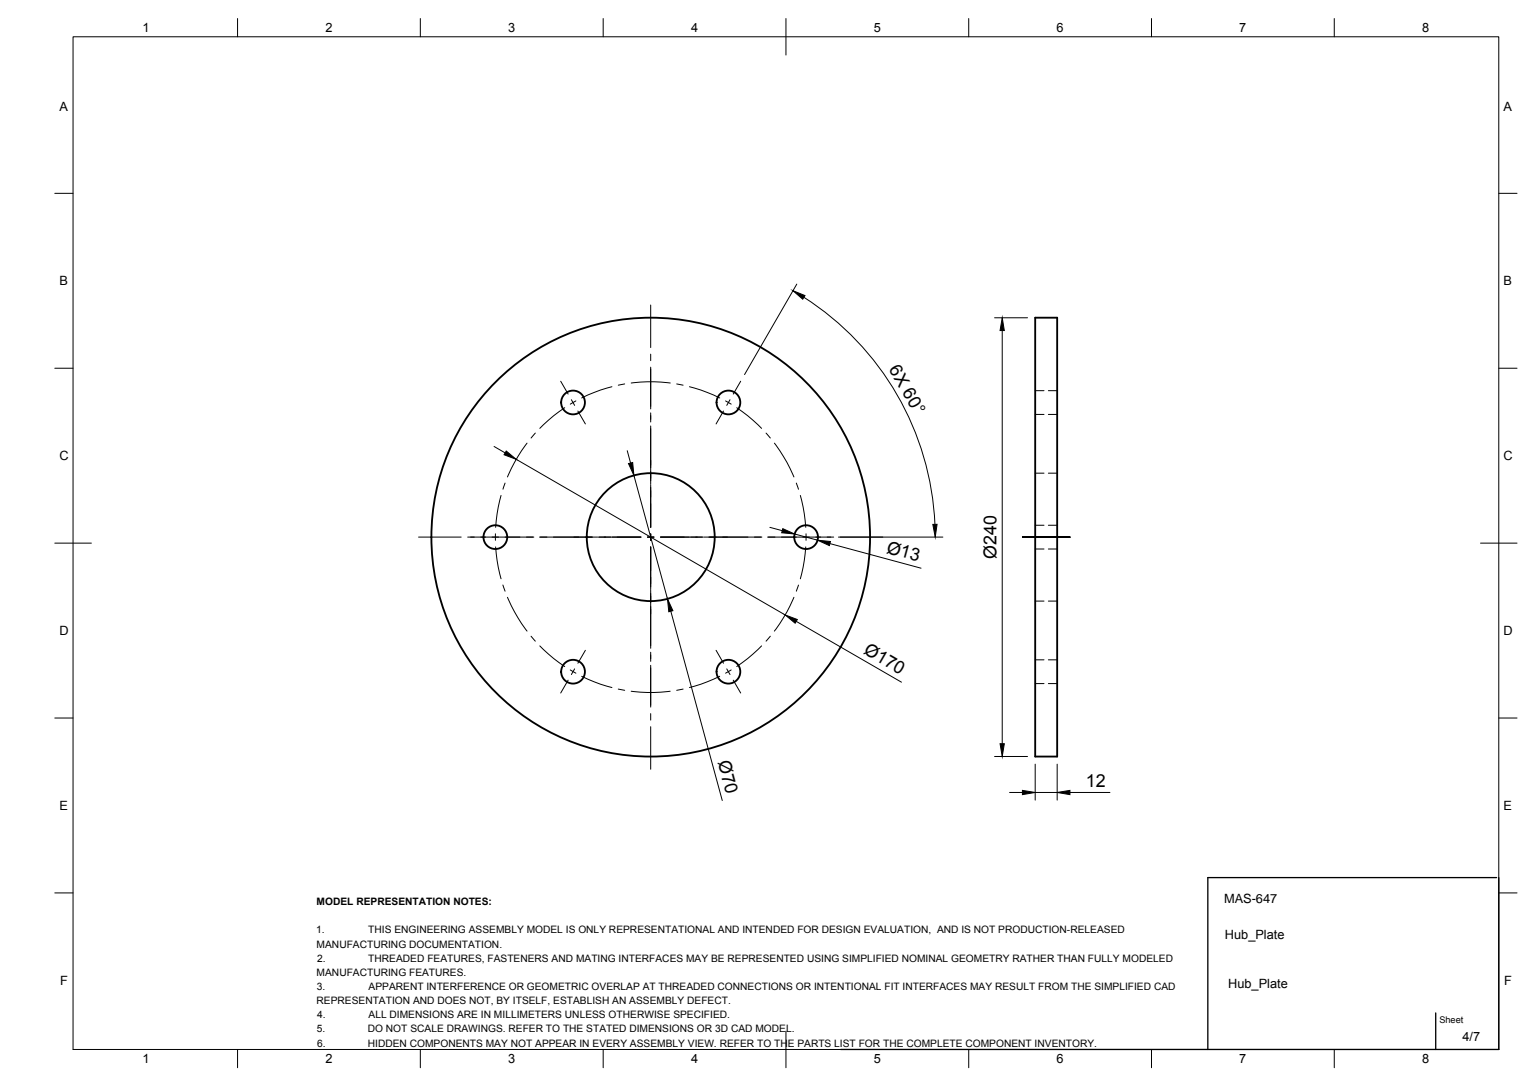
ISO-10303-21;
HEADER;
FILE_DESCRIPTION((''),'2;1');
FILE_NAME('Hub_Plate.step','2026-10-09T11:36:02-07:00',(''),(''),'','','');
FILE_SCHEMA (('AUTOMOTIVE_DESIGN { 1 0 10303 214 3 1 1 }'));
ENDSEC;
DATA;
#10=MECHANICAL_DESIGN_GEOMETRIC_PRESENTATION_REPRESENTATION('',(#83),#1549);
#73=SHAPE_REPRESENTATION_RELATIONSHIP('SRR','None',#1582,#78) ;
#78=ADVANCED_BREP_SHAPE_REPRESENTATION('',(#88),#1545) ;
#83=STYLED_ITEM('',(#1615),#88) ;
#88=MANIFOLD_SOLID_BREP('Body1',#845) ;
#106=FACE_BOUND('',#220,.T.) ;
#107=FACE_BOUND('',#221,.T.) ;
#108=FACE_BOUND('',#222,.T.) ;
#109=FACE_BOUND('',#223,.T.) ;
#110=FACE_BOUND('',#224,.T.) ;
#111=FACE_BOUND('',#225,.T.) ;
#112=FACE_BOUND('',#226,.T.) ;
#113=FACE_BOUND('',#228,.T.) ;
#114=FACE_BOUND('',#229,.T.) ;
#115=FACE_BOUND('',#230,.T.) ;
#116=FACE_BOUND('',#231,.T.) ;
#117=FACE_BOUND('',#232,.T.) ;
#118=FACE_BOUND('',#233,.T.) ;
#119=FACE_BOUND('',#234,.T.) ;
#125=PLANE('',#958) ;
#126=PLANE('',#959) ;
#151=FACE_OUTER_BOUND('',#211,.T.) ;
#152=FACE_OUTER_BOUND('',#212,.T.) ;
#153=FACE_OUTER_BOUND('',#213,.T.) ;
#154=FACE_OUTER_BOUND('',#214,.T.) ;
#155=FACE_OUTER_BOUND('',#215,.T.) ;
#156=FACE_OUTER_BOUND('',#216,.T.) ;
#157=FACE_OUTER_BOUND('',#217,.T.) ;
#158=FACE_OUTER_BOUND('',#218,.T.) ;
#159=FACE_OUTER_BOUND('',#219,.T.) ;
#160=FACE_OUTER_BOUND('',#227,.T.) ;
#211=EDGE_LOOP('',(#623,#624,#625,#626)) ;
#212=EDGE_LOOP('',(#627,#628,#629,#630)) ;
#213=EDGE_LOOP('',(#631,#632,#633,#634)) ;
#214=EDGE_LOOP('',(#635,#636,#637,#638)) ;
#215=EDGE_LOOP('',(#639,#640,#641,#642)) ;
#216=EDGE_LOOP('',(#643,#644,#645,#646)) ;
#217=EDGE_LOOP('',(#647,#648,#649,#650)) ;
#218=EDGE_LOOP('',(#651,#652,#653,#654)) ;
#219=EDGE_LOOP('',(#655)) ;
#220=EDGE_LOOP('',(#656)) ;
#221=EDGE_LOOP('',(#657)) ;
#222=EDGE_LOOP('',(#658)) ;
#223=EDGE_LOOP('',(#659)) ;
#224=EDGE_LOOP('',(#660)) ;
#225=EDGE_LOOP('',(#661)) ;
#226=EDGE_LOOP('',(#662)) ;
#227=EDGE_LOOP('',(#663)) ;
#228=EDGE_LOOP('',(#664)) ;
#229=EDGE_LOOP('',(#665)) ;
#230=EDGE_LOOP('',(#666)) ;
#231=EDGE_LOOP('',(#667)) ;
#232=EDGE_LOOP('',(#668)) ;
#233=EDGE_LOOP('',(#669)) ;
#234=EDGE_LOOP('',(#670)) ;
#272=LINE('',#1364,#320) ;
#273=LINE('',#1370,#321) ;
#274=LINE('',#1376,#322) ;
#275=LINE('',#1382,#323) ;
#276=LINE('',#1388,#324) ;
#277=LINE('',#1394,#325) ;
#278=LINE('',#1400,#326) ;
#279=LINE('',#1406,#327) ;
#320=VECTOR('',#1093,6.49999999999999) ;
#321=VECTOR('',#1100,6.49999999999999) ;
#322=VECTOR('',#1107,6.49999999999999) ;
#323=VECTOR('',#1114,6.49999999999999) ;
#324=VECTOR('',#1121,6.49999999999999) ;
#325=VECTOR('',#1128,6.49999999999999) ;
#326=VECTOR('',#1135,35.) ;
#327=VECTOR('',#1142,120.) ;
#376=CIRCLE('',#935,6.49999999999999) ;
#377=CIRCLE('',#936,6.49999999999999) ;
#378=CIRCLE('',#938,6.49999999999999) ;
#379=CIRCLE('',#939,6.49999999999998) ;
#380=CIRCLE('',#941,6.49999999999999) ;
#381=CIRCLE('',#942,6.49999999999999) ;
#382=CIRCLE('',#944,6.49999999999999) ;
#383=CIRCLE('',#945,6.49999999999999) ;
#384=CIRCLE('',#947,6.49999999999999) ;
#385=CIRCLE('',#948,6.49999999999999) ;
#386=CIRCLE('',#950,6.49999999999999) ;
#387=CIRCLE('',#951,6.49999999999999) ;
#388=CIRCLE('',#953,35.) ;
#389=CIRCLE('',#954,35.) ;
#390=CIRCLE('',#956,120.) ;
#391=CIRCLE('',#957,120.) ;
#428=VERTEX_POINT('',#1361) ;
#429=VERTEX_POINT('',#1363) ;
#430=VERTEX_POINT('',#1367) ;
#431=VERTEX_POINT('',#1369) ;
#432=VERTEX_POINT('',#1373) ;
#433=VERTEX_POINT('',#1375) ;
#434=VERTEX_POINT('',#1379) ;
#435=VERTEX_POINT('',#1381) ;
#436=VERTEX_POINT('',#1385) ;
#437=VERTEX_POINT('',#1387) ;
#438=VERTEX_POINT('',#1391) ;
#439=VERTEX_POINT('',#1393) ;
#440=VERTEX_POINT('',#1397) ;
#441=VERTEX_POINT('',#1399) ;
#442=VERTEX_POINT('',#1403) ;
#443=VERTEX_POINT('',#1405) ;
#499=EDGE_CURVE('',#428,#428,#376,.T.) ;
#500=EDGE_CURVE('',#428,#429,#272,.T.) ;
#501=EDGE_CURVE('',#429,#429,#377,.T.) ;
#502=EDGE_CURVE('',#430,#430,#378,.T.) ;
#503=EDGE_CURVE('',#430,#431,#273,.T.) ;
#504=EDGE_CURVE('',#431,#431,#379,.T.) ;
#505=EDGE_CURVE('',#432,#432,#380,.T.) ;
#506=EDGE_CURVE('',#432,#433,#274,.T.) ;
#507=EDGE_CURVE('',#433,#433,#381,.T.) ;
#508=EDGE_CURVE('',#434,#434,#382,.T.) ;
#509=EDGE_CURVE('',#434,#435,#275,.T.) ;
#510=EDGE_CURVE('',#435,#435,#383,.T.) ;
#511=EDGE_CURVE('',#436,#436,#384,.T.) ;
#512=EDGE_CURVE('',#436,#437,#276,.T.) ;
#513=EDGE_CURVE('',#437,#437,#385,.T.) ;
#514=EDGE_CURVE('',#438,#438,#386,.T.) ;
#515=EDGE_CURVE('',#438,#439,#277,.T.) ;
#516=EDGE_CURVE('',#439,#439,#387,.T.) ;
#517=EDGE_CURVE('',#440,#440,#388,.T.) ;
#518=EDGE_CURVE('',#440,#441,#278,.T.) ;
#519=EDGE_CURVE('',#441,#441,#389,.T.) ;
#520=EDGE_CURVE('',#442,#442,#390,.T.) ;
#521=EDGE_CURVE('',#442,#443,#279,.T.) ;
#522=EDGE_CURVE('',#443,#443,#391,.T.) ;
#623=ORIENTED_EDGE('',*,*,#499,.F.) ;
#624=ORIENTED_EDGE('',*,*,#500,.T.) ;
#625=ORIENTED_EDGE('',*,*,#501,.T.) ;
#626=ORIENTED_EDGE('',*,*,#500,.F.) ;
#627=ORIENTED_EDGE('',*,*,#502,.F.) ;
#628=ORIENTED_EDGE('',*,*,#503,.T.) ;
#629=ORIENTED_EDGE('',*,*,#504,.T.) ;
#630=ORIENTED_EDGE('',*,*,#503,.F.) ;
#631=ORIENTED_EDGE('',*,*,#505,.F.) ;
#632=ORIENTED_EDGE('',*,*,#506,.T.) ;
#633=ORIENTED_EDGE('',*,*,#507,.T.) ;
#634=ORIENTED_EDGE('',*,*,#506,.F.) ;
#635=ORIENTED_EDGE('',*,*,#508,.F.) ;
#636=ORIENTED_EDGE('',*,*,#509,.T.) ;
#637=ORIENTED_EDGE('',*,*,#510,.T.) ;
#638=ORIENTED_EDGE('',*,*,#509,.F.) ;
#639=ORIENTED_EDGE('',*,*,#511,.F.) ;
#640=ORIENTED_EDGE('',*,*,#512,.T.) ;
#641=ORIENTED_EDGE('',*,*,#513,.T.) ;
#642=ORIENTED_EDGE('',*,*,#512,.F.) ;
#643=ORIENTED_EDGE('',*,*,#514,.F.) ;
#644=ORIENTED_EDGE('',*,*,#515,.T.) ;
#645=ORIENTED_EDGE('',*,*,#516,.T.) ;
#646=ORIENTED_EDGE('',*,*,#515,.F.) ;
#647=ORIENTED_EDGE('',*,*,#517,.T.) ;
#648=ORIENTED_EDGE('',*,*,#518,.T.) ;
#649=ORIENTED_EDGE('',*,*,#519,.F.) ;
#650=ORIENTED_EDGE('',*,*,#518,.F.) ;
#651=ORIENTED_EDGE('',*,*,#520,.T.) ;
#652=ORIENTED_EDGE('',*,*,#521,.T.) ;
#653=ORIENTED_EDGE('',*,*,#522,.F.) ;
#654=ORIENTED_EDGE('',*,*,#521,.F.) ;
#655=ORIENTED_EDGE('',*,*,#522,.T.) ;
#656=ORIENTED_EDGE('',*,*,#517,.F.) ;
#657=ORIENTED_EDGE('',*,*,#501,.F.) ;
#658=ORIENTED_EDGE('',*,*,#504,.F.) ;
#659=ORIENTED_EDGE('',*,*,#507,.F.) ;
#660=ORIENTED_EDGE('',*,*,#510,.F.) ;
#661=ORIENTED_EDGE('',*,*,#513,.F.) ;
#662=ORIENTED_EDGE('',*,*,#516,.F.) ;
#663=ORIENTED_EDGE('',*,*,#520,.F.) ;
#664=ORIENTED_EDGE('',*,*,#519,.T.) ;
#665=ORIENTED_EDGE('',*,*,#499,.T.) ;
#666=ORIENTED_EDGE('',*,*,#502,.T.) ;
#667=ORIENTED_EDGE('',*,*,#505,.T.) ;
#668=ORIENTED_EDGE('',*,*,#508,.T.) ;
#669=ORIENTED_EDGE('',*,*,#511,.T.) ;
#670=ORIENTED_EDGE('',*,*,#514,.T.) ;
#783=CYLINDRICAL_SURFACE('',#934,6.49999999999999) ;
#784=CYLINDRICAL_SURFACE('',#937,6.49999999999999) ;
#785=CYLINDRICAL_SURFACE('',#940,6.49999999999999) ;
#786=CYLINDRICAL_SURFACE('',#943,6.49999999999999) ;
#787=CYLINDRICAL_SURFACE('',#946,6.49999999999999) ;
#788=CYLINDRICAL_SURFACE('',#949,6.49999999999999) ;
#789=CYLINDRICAL_SURFACE('',#952,35.) ;
#790=CYLINDRICAL_SURFACE('',#955,120.) ;
#808=ADVANCED_FACE('',(#151),#783,.F.) ;
#809=ADVANCED_FACE('',(#152),#784,.F.) ;
#810=ADVANCED_FACE('',(#153),#785,.F.) ;
#811=ADVANCED_FACE('',(#154),#786,.F.) ;
#812=ADVANCED_FACE('',(#155),#787,.F.) ;
#813=ADVANCED_FACE('',(#156),#788,.F.) ;
#814=ADVANCED_FACE('',(#157),#789,.F.) ;
#815=ADVANCED_FACE('',(#158),#790,.T.) ;
#816=ADVANCED_FACE('',(#159,#106,#107,#108,#109,#110,#111,#112),#125,.T.) ;
#817=ADVANCED_FACE('',(#160,#113,#114,#115,#116,#117,#118,#119),#126,.F.) ;
#845=CLOSED_SHELL('',(#808,#809,#810,#811,#812,#813,#814,#815,#816,#817)) ;
#933=AXIS2_PLACEMENT_3D('',#1359,#1087,#1088) ;
#934=AXIS2_PLACEMENT_3D('',#1360,#1089,#1090) ;
#935=AXIS2_PLACEMENT_3D('',#1362,#1091,#1092) ;
#936=AXIS2_PLACEMENT_3D('',#1365,#1094,#1095) ;
#937=AXIS2_PLACEMENT_3D('',#1366,#1096,#1097) ;
#938=AXIS2_PLACEMENT_3D('',#1368,#1098,#1099) ;
#939=AXIS2_PLACEMENT_3D('',#1371,#1101,#1102) ;
#940=AXIS2_PLACEMENT_3D('',#1372,#1103,#1104) ;
#941=AXIS2_PLACEMENT_3D('',#1374,#1105,#1106) ;
#942=AXIS2_PLACEMENT_3D('',#1377,#1108,#1109) ;
#943=AXIS2_PLACEMENT_3D('',#1378,#1110,#1111) ;
#944=AXIS2_PLACEMENT_3D('',#1380,#1112,#1113) ;
#945=AXIS2_PLACEMENT_3D('',#1383,#1115,#1116) ;
#946=AXIS2_PLACEMENT_3D('',#1384,#1117,#1118) ;
#947=AXIS2_PLACEMENT_3D('',#1386,#1119,#1120) ;
#948=AXIS2_PLACEMENT_3D('',#1389,#1122,#1123) ;
#949=AXIS2_PLACEMENT_3D('',#1390,#1124,#1125) ;
#950=AXIS2_PLACEMENT_3D('',#1392,#1126,#1127) ;
#951=AXIS2_PLACEMENT_3D('',#1395,#1129,#1130) ;
#952=AXIS2_PLACEMENT_3D('',#1396,#1131,#1132) ;
#953=AXIS2_PLACEMENT_3D('',#1398,#1133,#1134) ;
#954=AXIS2_PLACEMENT_3D('',#1401,#1136,#1137) ;
#955=AXIS2_PLACEMENT_3D('',#1402,#1138,#1139) ;
#956=AXIS2_PLACEMENT_3D('',#1404,#1140,#1141) ;
#957=AXIS2_PLACEMENT_3D('',#1407,#1143,#1144) ;
#958=AXIS2_PLACEMENT_3D('',#1408,#1145,#1146) ;
#959=AXIS2_PLACEMENT_3D('',#1409,#1147,#1148) ;
#1087=DIRECTION('axis',(0.,0.,1.)) ;
#1088=DIRECTION('refdir',(1.,0.,0.)) ;
#1089=DIRECTION('center_axis',(1.,0.,0.)) ;
#1090=DIRECTION('ref_axis',(0.,0.,-1.)) ;
#1091=DIRECTION('center_axis',(1.,0.,0.)) ;
#1092=DIRECTION('ref_axis',(0.,0.,-1.)) ;
#1093=DIRECTION('',(1.,0.,0.)) ;
#1094=DIRECTION('center_axis',(1.,0.,0.)) ;
#1095=DIRECTION('ref_axis',(0.,0.,-1.)) ;
#1096=DIRECTION('center_axis',(1.,0.,0.)) ;
#1097=DIRECTION('ref_axis',(0.,0.,-1.)) ;
#1098=DIRECTION('center_axis',(1.,0.,0.)) ;
#1099=DIRECTION('ref_axis',(0.,0.,-1.)) ;
#1100=DIRECTION('',(1.,0.,0.)) ;
#1101=DIRECTION('center_axis',(1.,0.,0.)) ;
#1102=DIRECTION('ref_axis',(0.,0.,-1.)) ;
#1103=DIRECTION('center_axis',(1.,0.,0.)) ;
#1104=DIRECTION('ref_axis',(0.,0.,-1.)) ;
#1105=DIRECTION('center_axis',(1.,0.,0.)) ;
#1106=DIRECTION('ref_axis',(0.,0.,-1.)) ;
#1107=DIRECTION('',(1.,0.,0.)) ;
#1108=DIRECTION('center_axis',(1.,0.,0.)) ;
#1109=DIRECTION('ref_axis',(0.,0.,-1.)) ;
#1110=DIRECTION('center_axis',(1.,0.,0.)) ;
#1111=DIRECTION('ref_axis',(0.,0.,-1.)) ;
#1112=DIRECTION('center_axis',(1.,0.,0.)) ;
#1113=DIRECTION('ref_axis',(0.,0.,-1.)) ;
#1114=DIRECTION('',(1.,0.,0.)) ;
#1115=DIRECTION('center_axis',(1.,0.,0.)) ;
#1116=DIRECTION('ref_axis',(0.,0.,-1.)) ;
#1117=DIRECTION('center_axis',(1.,0.,0.)) ;
#1118=DIRECTION('ref_axis',(0.,0.,-1.)) ;
#1119=DIRECTION('center_axis',(1.,0.,0.)) ;
#1120=DIRECTION('ref_axis',(0.,0.,-1.)) ;
#1121=DIRECTION('',(1.,0.,0.)) ;
#1122=DIRECTION('center_axis',(1.,0.,0.)) ;
#1123=DIRECTION('ref_axis',(0.,0.,-1.)) ;
#1124=DIRECTION('center_axis',(1.,0.,0.)) ;
#1125=DIRECTION('ref_axis',(0.,0.,-1.)) ;
#1126=DIRECTION('center_axis',(1.,0.,0.)) ;
#1127=DIRECTION('ref_axis',(0.,0.,-1.)) ;
#1128=DIRECTION('',(1.,0.,0.)) ;
#1129=DIRECTION('center_axis',(1.,0.,0.)) ;
#1130=DIRECTION('ref_axis',(0.,0.,-1.)) ;
#1131=DIRECTION('center_axis',(-1.,0.,0.)) ;
#1132=DIRECTION('ref_axis',(0.,0.,1.)) ;
#1133=DIRECTION('center_axis',(1.,0.,0.)) ;
#1134=DIRECTION('ref_axis',(0.,0.,-1.)) ;
#1135=DIRECTION('',(-1.,0.,0.)) ;
#1136=DIRECTION('center_axis',(1.,0.,0.)) ;
#1137=DIRECTION('ref_axis',(0.,0.,-1.)) ;
#1138=DIRECTION('center_axis',(-1.,0.,0.)) ;
#1139=DIRECTION('ref_axis',(0.,0.,1.)) ;
#1140=DIRECTION('center_axis',(1.,0.,0.)) ;
#1141=DIRECTION('ref_axis',(0.,0.,-1.)) ;
#1142=DIRECTION('',(1.,0.,0.)) ;
#1143=DIRECTION('center_axis',(1.,0.,0.)) ;
#1144=DIRECTION('ref_axis',(0.,0.,-1.)) ;
#1145=DIRECTION('center_axis',(1.,0.,0.)) ;
#1146=DIRECTION('ref_axis',(0.,0.,-1.)) ;
#1147=DIRECTION('center_axis',(1.,0.,0.)) ;
#1148=DIRECTION('ref_axis',(0.,0.,-1.)) ;
#1359=CARTESIAN_POINT('',(0.,0.,0.)) ;
#1360=CARTESIAN_POINT('Origin',(12.,42.5000000000009,-73.6121593216768)) ;
#1361=CARTESIAN_POINT('',(4.44089209850063E-15,42.5000000000009,-67.1121593216768)) ;
#1362=CARTESIAN_POINT('Origin',(3.46944695195361E-15,42.5000000000009,-73.6121593216768)) ;
#1363=CARTESIAN_POINT('',(12.,42.5000000000009,-67.1121593216768)) ;
#1364=CARTESIAN_POINT('',(12.,42.5000000000009,-67.1121593216768)) ;
#1365=CARTESIAN_POINT('Origin',(12.,42.5000000000009,-73.6121593216768)) ;
#1366=CARTESIAN_POINT('Origin',(12.,-42.4999999999993,-73.6121593216777)) ;
#1367=CARTESIAN_POINT('',(4.44089209850063E-15,-42.4999999999993,-67.1121593216777)) ;
#1368=CARTESIAN_POINT('Origin',(3.46944695195361E-15,-42.4999999999993,
-73.6121593216777)) ;
#1369=CARTESIAN_POINT('',(12.,-42.4999999999993,-67.1121593216777)) ;
#1370=CARTESIAN_POINT('',(12.,-42.4999999999993,-67.1121593216777)) ;
#1371=CARTESIAN_POINT('Origin',(12.,-42.4999999999993,-73.6121593216777)) ;
#1372=CARTESIAN_POINT('Origin',(12.,-85.,0.)) ;
#1373=CARTESIAN_POINT('',(4.44089209850063E-15,-85.,6.49999999999999)) ;
#1374=CARTESIAN_POINT('Origin',(3.46944695195361E-15,-85.,0.)) ;
#1375=CARTESIAN_POINT('',(12.,-85.,6.49999999999999)) ;
#1376=CARTESIAN_POINT('',(12.,-85.,6.49999999999999)) ;
#1377=CARTESIAN_POINT('Origin',(12.,-85.,0.)) ;
#1378=CARTESIAN_POINT('Origin',(12.,-42.5000000000003,73.6121593216771)) ;
#1379=CARTESIAN_POINT('',(4.44089209850063E-15,-42.5000000000003,80.1121593216771)) ;
#1380=CARTESIAN_POINT('Origin',(3.46944695195361E-15,-42.5000000000003,
73.6121593216771)) ;
#1381=CARTESIAN_POINT('',(12.,-42.5000000000003,80.1121593216771)) ;
#1382=CARTESIAN_POINT('',(12.,-42.5000000000003,80.1121593216771)) ;
#1383=CARTESIAN_POINT('Origin',(12.,-42.5000000000003,73.6121593216771)) ;
#1384=CARTESIAN_POINT('Origin',(12.,42.4999999999998,73.6121593216774)) ;
#1385=CARTESIAN_POINT('',(4.44089209850063E-15,42.4999999999998,80.1121593216774)) ;
#1386=CARTESIAN_POINT('Origin',(3.46944695195361E-15,42.4999999999998,73.6121593216774)) ;
#1387=CARTESIAN_POINT('',(12.,42.4999999999998,80.1121593216774)) ;
#1388=CARTESIAN_POINT('',(12.,42.4999999999998,80.1121593216774)) ;
#1389=CARTESIAN_POINT('Origin',(12.,42.4999999999998,73.6121593216774)) ;
#1390=CARTESIAN_POINT('Origin',(12.,85.,0.)) ;
#1391=CARTESIAN_POINT('',(4.44089209850063E-15,85.,6.49999999999999)) ;
#1392=CARTESIAN_POINT('Origin',(3.46944695195361E-15,85.,0.)) ;
#1393=CARTESIAN_POINT('',(12.,85.,6.49999999999999)) ;
#1394=CARTESIAN_POINT('',(12.,85.,6.49999999999999)) ;
#1395=CARTESIAN_POINT('Origin',(12.,85.,0.)) ;
#1396=CARTESIAN_POINT('Origin',(12.,0.,0.)) ;
#1397=CARTESIAN_POINT('',(12.,-4.28626379701574E-15,-35.)) ;
#1398=CARTESIAN_POINT('Origin',(12.,0.,0.)) ;
#1399=CARTESIAN_POINT('',(0.,-4.28626379701574E-15,-35.)) ;
#1400=CARTESIAN_POINT('',(12.,-4.28626379701574E-15,-35.)) ;
#1401=CARTESIAN_POINT('Origin',(0.,0.,0.)) ;
#1402=CARTESIAN_POINT('Origin',(12.,0.,0.)) ;
#1403=CARTESIAN_POINT('',(0.,-1.46957615897682E-14,-120.)) ;
#1404=CARTESIAN_POINT('Origin',(0.,0.,0.)) ;
#1405=CARTESIAN_POINT('',(12.,-1.46957615897682E-14,-120.)) ;
#1406=CARTESIAN_POINT('',(12.,-1.46957615897682E-14,-120.)) ;
#1407=CARTESIAN_POINT('Origin',(12.,0.,0.)) ;
#1408=CARTESIAN_POINT('Origin',(12.,0.,0.)) ;
#1409=CARTESIAN_POINT('Origin',(0.,0.,0.)) ;
#1538=UNCERTAINTY_MEASURE_WITH_UNIT(LENGTH_MEASURE(0.01),#1550,
'DISTANCE_ACCURACY_VALUE',
'Maximum model space distance between geometric entities at asserted c
onnectivities') ;
#1542=UNCERTAINTY_MEASURE_WITH_UNIT(LENGTH_MEASURE(0.01),#1550,
'DISTANCE_ACCURACY_VALUE',
'Maximum model space distance between geometric entities at asserted c
onnectivities') ;
#1545=(
GEOMETRIC_REPRESENTATION_CONTEXT(3)
GLOBAL_UNCERTAINTY_ASSIGNED_CONTEXT((#1538))
GLOBAL_UNIT_ASSIGNED_CONTEXT((#1550,#1552,#1553))
REPRESENTATION_CONTEXT('','3D')
) ;
#1549=(
GEOMETRIC_REPRESENTATION_CONTEXT(3)
GLOBAL_UNCERTAINTY_ASSIGNED_CONTEXT((#1542))
GLOBAL_UNIT_ASSIGNED_CONTEXT((#1550,#1552,#1553))
REPRESENTATION_CONTEXT('','3D')
) ;
#1550=(
LENGTH_UNIT()
NAMED_UNIT(*)
SI_UNIT(.MILLI.,.METRE.)
) ;
#1552=(
NAMED_UNIT(*)
PLANE_ANGLE_UNIT()
SI_UNIT($,.RADIAN.)
) ;
#1553=(
NAMED_UNIT(*)
SI_UNIT($,.STERADIAN.)
SOLID_ANGLE_UNIT()
) ;
#1556=SHAPE_DEFINITION_REPRESENTATION(#1562,#1582) ;
#1562=PRODUCT_DEFINITION_SHAPE('',$,#1589) ;
#1582=SHAPE_REPRESENTATION('',(#933),#1545) ;
#1586=PRODUCT_DEFINITION_CONTEXT('part definition',#1606,'design') ;
#1589=PRODUCT_DEFINITION('Hub_Plate','Hub_Plate',#1595,#1586) ;
#1595=PRODUCT_DEFINITION_FORMATION('',$,#1610) ;
#1606=APPLICATION_CONTEXT(
'Core Data for Automotive Mechanical Design Process') ;
#1607=PRODUCT_CONTEXT('part definition',#1606,'mechanical') ;
#1610=PRODUCT('Hub_Plate','Hub_Plate',$,(#1607)) ;
#1615=PRESENTATION_STYLE_ASSIGNMENT((#1617)) ;
#1617=SURFACE_STYLE_USAGE(.BOTH.,#1619) ;
#1619=SURFACE_SIDE_STYLE('',(#1621)) ;
#1621=SURFACE_STYLE_FILL_AREA(#1623) ;
#1623=FILL_AREA_STYLE('Opaque(202,209,238)',(#1625)) ;
#1625=FILL_AREA_STYLE_COLOUR('Opaque(202,209,238)',#1627) ;
#1627=COLOUR_RGB('Opaque(202,209,238)', 0.09019608, 0.27058824, 0.51372549) ;
ENDSEC;
END-ISO-10303-21;
